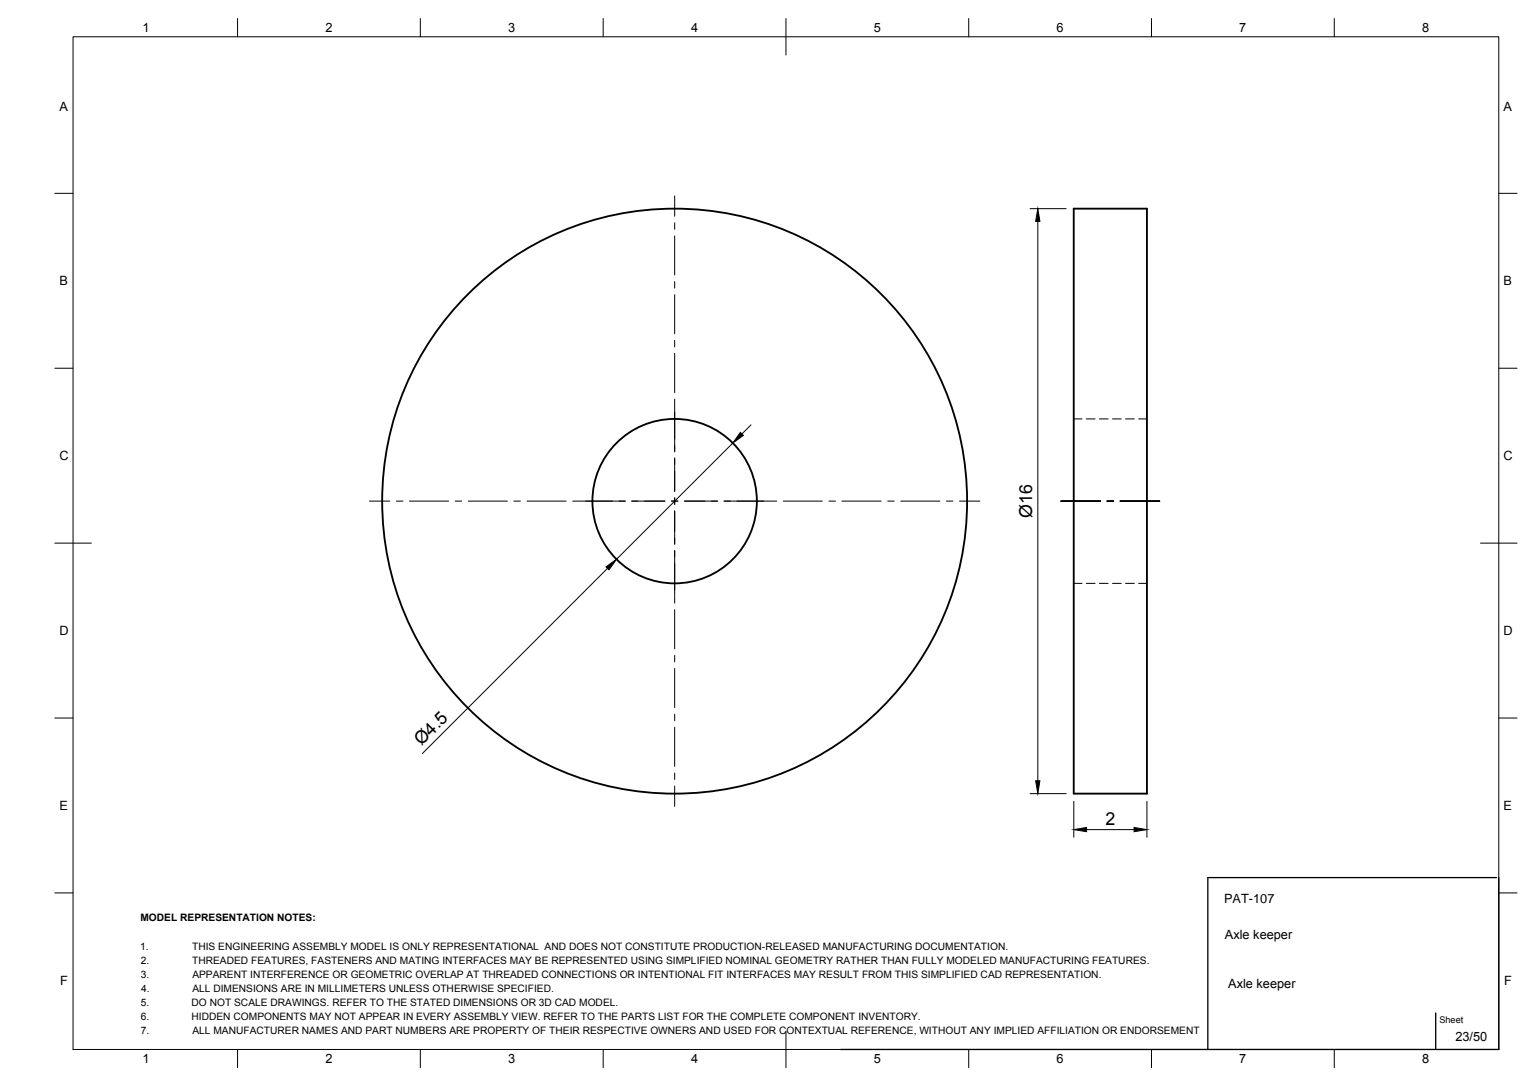
ISO-10303-21;
HEADER;
/* Generated by software containing ST-Developer
 * from STEP Tools, Inc. (www.steptools.com) 
 */

FILE_DESCRIPTION(
/* description */ ('Turntable on roller ring'),
/* implementation_level */ '2;1');

FILE_NAME(
/* name */ 'Axle keeper.step',
/* time_stamp */ '2026-10-28T03:23:59-07:00',
/* author */ (''),
/* organization */ (''),
/* preprocessor_version */ 'ST-DEVELOPER v20.2',
/* originating_system */ 'Autodesk Translation Framework v15.17.0.0',
/* authorisation */ '');

FILE_SCHEMA (('AUTOMOTIVE_DESIGN { 1 0 10303 214 3 1 1 }'));
ENDSEC;

DATA;
#10=MECHANICAL_DESIGN_GEOMETRIC_PRESENTATION_REPRESENTATION('',(#646),#16281);
#527=SHAPE_REPRESENTATION_RELATIONSHIP('SRR','None',#16544,#582);
#582=ADVANCED_BREP_SHAPE_REPRESENTATION('',(#716),#16238);
#646=STYLED_ITEM('',(#16932),#716);
#716=MANIFOLD_SOLID_BREP('Body1',#8389);
#887=FACE_BOUND('',#2135,.T.);
#888=FACE_BOUND('',#2137,.T.);
#1107=PLANE('',#9607);
#1108=PLANE('',#9608);
#1497=FACE_OUTER_BOUND('',#2132,.T.);
#1498=FACE_OUTER_BOUND('',#2133,.T.);
#1499=FACE_OUTER_BOUND('',#2134,.T.);
#1500=FACE_OUTER_BOUND('',#2136,.T.);
#2132=EDGE_LOOP('',(#6695,#6696,#6697,#6698));
#2133=EDGE_LOOP('',(#6699,#6700,#6701,#6702));
#2134=EDGE_LOOP('',(#6703));
#2135=EDGE_LOOP('',(#6704));
#2136=EDGE_LOOP('',(#6705));
#2137=EDGE_LOOP('',(#6706));
#2735=LINE('',#14620,#3218);
#2736=LINE('',#14626,#3219);
#3218=VECTOR('',#11568,0.225);
#3219=VECTOR('',#11575,0.8);
#3721=CIRCLE('',#9602,0.225);
#3722=CIRCLE('',#9603,0.225);
#3723=CIRCLE('',#9605,0.8);
#3724=CIRCLE('',#9606,0.8);
#4301=VERTEX_POINT('',#14617);
#4302=VERTEX_POINT('',#14619);
#4303=VERTEX_POINT('',#14623);
#4304=VERTEX_POINT('',#14625);
#5158=EDGE_CURVE('',#4301,#4301,#3721,.T.);
#5159=EDGE_CURVE('',#4301,#4302,#2735,.T.);
#5160=EDGE_CURVE('',#4302,#4302,#3722,.T.);
#5161=EDGE_CURVE('',#4303,#4303,#3723,.T.);
#5162=EDGE_CURVE('',#4303,#4304,#2736,.T.);
#5163=EDGE_CURVE('',#4304,#4304,#3724,.T.);
#6695=ORIENTED_EDGE('',*,*,#5158,.F.);
#6696=ORIENTED_EDGE('',*,*,#5159,.T.);
#6697=ORIENTED_EDGE('',*,*,#5160,.T.);
#6698=ORIENTED_EDGE('',*,*,#5159,.F.);
#6699=ORIENTED_EDGE('',*,*,#5161,.F.);
#6700=ORIENTED_EDGE('',*,*,#5162,.T.);
#6701=ORIENTED_EDGE('',*,*,#5163,.T.);
#6702=ORIENTED_EDGE('',*,*,#5162,.F.);
#6703=ORIENTED_EDGE('',*,*,#5161,.T.);
#6704=ORIENTED_EDGE('',*,*,#5158,.T.);
#6705=ORIENTED_EDGE('',*,*,#5163,.F.);
#6706=ORIENTED_EDGE('',*,*,#5160,.F.);
#7766=CYLINDRICAL_SURFACE('',#9601,0.225);
#7767=CYLINDRICAL_SURFACE('',#9604,0.8);
#8100=ADVANCED_FACE('',(#1497),#7766,.F.);
#8101=ADVANCED_FACE('',(#1498),#7767,.T.);
#8102=ADVANCED_FACE('',(#1499,#887),#1107,.T.);
#8103=ADVANCED_FACE('',(#1500,#888),#1108,.F.);
#8389=CLOSED_SHELL('',(#8100,#8101,#8102,#8103));
#9600=AXIS2_PLACEMENT_3D('',#14615,#11562,#11563);
#9601=AXIS2_PLACEMENT_3D('',#14616,#11564,#11565);
#9602=AXIS2_PLACEMENT_3D('',#14618,#11566,#11567);
#9603=AXIS2_PLACEMENT_3D('',#14621,#11569,#11570);
#9604=AXIS2_PLACEMENT_3D('',#14622,#11571,#11572);
#9605=AXIS2_PLACEMENT_3D('',#14624,#11573,#11574);
#9606=AXIS2_PLACEMENT_3D('',#14627,#11576,#11577);
#9607=AXIS2_PLACEMENT_3D('',#14628,#11578,#11579);
#9608=AXIS2_PLACEMENT_3D('',#14629,#11580,#11581);
#11562=DIRECTION('axis',(0.,0.,1.));
#11563=DIRECTION('refdir',(1.,0.,0.));
#11564=DIRECTION('center_axis',(0.,1.,0.));
#11565=DIRECTION('ref_axis',(1.,0.,0.));
#11566=DIRECTION('center_axis',(0.,-1.,0.));
#11567=DIRECTION('ref_axis',(1.,0.,0.));
#11568=DIRECTION('',(0.,-1.,0.));
#11569=DIRECTION('center_axis',(0.,-1.,0.));
#11570=DIRECTION('ref_axis',(1.,0.,0.));
#11571=DIRECTION('center_axis',(0.,1.,0.));
#11572=DIRECTION('ref_axis',(1.,0.,0.));
#11573=DIRECTION('center_axis',(0.,1.,0.));
#11574=DIRECTION('ref_axis',(1.,0.,0.));
#11575=DIRECTION('',(0.,-1.,0.));
#11576=DIRECTION('center_axis',(0.,1.,0.));
#11577=DIRECTION('ref_axis',(1.,0.,0.));
#11578=DIRECTION('center_axis',(0.,1.,0.));
#11579=DIRECTION('ref_axis',(1.,0.,0.));
#11580=DIRECTION('center_axis',(0.,1.,0.));
#11581=DIRECTION('ref_axis',(1.,0.,0.));
#14615=CARTESIAN_POINT('',(0.,0.,0.));
#14616=CARTESIAN_POINT('Origin',(0.,16.3,3.5));
#14617=CARTESIAN_POINT('',(-0.225,16.5,3.5));
#14618=CARTESIAN_POINT('Origin',(0.,16.5,3.5));
#14619=CARTESIAN_POINT('',(-0.225,16.3,3.5));
#14620=CARTESIAN_POINT('',(-0.225,16.3,3.5));
#14621=CARTESIAN_POINT('Origin',(0.,16.3,3.5));
#14622=CARTESIAN_POINT('Origin',(0.,16.3,3.5));
#14623=CARTESIAN_POINT('',(-0.8,16.5,3.5));
#14624=CARTESIAN_POINT('Origin',(0.,16.5,3.5));
#14625=CARTESIAN_POINT('',(-0.8,16.3,3.5));
#14626=CARTESIAN_POINT('',(-0.8,16.3,3.5));
#14627=CARTESIAN_POINT('Origin',(0.,16.3,3.5));
#14628=CARTESIAN_POINT('Origin',(0.,16.5,3.5));
#14629=CARTESIAN_POINT('Origin',(0.,16.3,3.5));
#16169=UNCERTAINTY_MEASURE_WITH_UNIT(LENGTH_MEASURE(0.001),#16282,
'DISTANCE_ACCURACY_VALUE',
'Maximum model space distance between geometric entities at asserted c
onnectivities');
#16212=UNCERTAINTY_MEASURE_WITH_UNIT(LENGTH_MEASURE(0.001),#16282,
'DISTANCE_ACCURACY_VALUE',
'Maximum model space distance between geometric entities at asserted c
onnectivities');
#16238=(
GEOMETRIC_REPRESENTATION_CONTEXT(3)
GLOBAL_UNCERTAINTY_ASSIGNED_CONTEXT((#16169))
GLOBAL_UNIT_ASSIGNED_CONTEXT((#16282,#16284,#16285))
REPRESENTATION_CONTEXT('','3D')
);
#16281=(
GEOMETRIC_REPRESENTATION_CONTEXT(3)
GLOBAL_UNCERTAINTY_ASSIGNED_CONTEXT((#16212))
GLOBAL_UNIT_ASSIGNED_CONTEXT((#16282,#16284,#16285))
REPRESENTATION_CONTEXT('','3D')
);
#16282=(
LENGTH_UNIT()
NAMED_UNIT(*)
SI_UNIT(.CENTI.,.METRE.)
);
#16284=(
NAMED_UNIT(*)
PLANE_ANGLE_UNIT()
SI_UNIT($,.RADIAN.)
);
#16285=(
NAMED_UNIT(*)
SI_UNIT($,.STERADIAN.)
SOLID_ANGLE_UNIT()
);
#16311=SHAPE_DEFINITION_REPRESENTATION(#16405,#16544);
#16405=PRODUCT_DEFINITION_SHAPE('',$,#16613);
#16544=SHAPE_REPRESENTATION('',(#9600),#16238);
#16587=PRODUCT_DEFINITION_CONTEXT('part definition',#16793,'design');
#16613=PRODUCT_DEFINITION('Axle keeper','Axle keeper',#16681,#16587);
#16681=PRODUCT_DEFINITION_FORMATION('',$,#16820);
#16793=APPLICATION_CONTEXT(
'Core Data for Automotive Mechanical Design Process');
#16794=PRODUCT_CONTEXT('part definition',#16793,'mechanical');
#16820=PRODUCT('Axle keeper','Axle keeper','Axle keeper',(#16794));
#16926=COLOUR_RGB('Grey',0.48,0.52,0.57);
#16927=FILL_AREA_STYLE_COLOUR('',#16926);
#16928=FILL_AREA_STYLE('',(#16927));
#16929=SURFACE_STYLE_FILL_AREA(#16928);
#16930=SURFACE_SIDE_STYLE('',(#16929));
#16931=SURFACE_STYLE_USAGE(.BOTH.,#16930);
#16932=PRESENTATION_STYLE_ASSIGNMENT((#16931));
ENDSEC;
END-ISO-10303-21;
